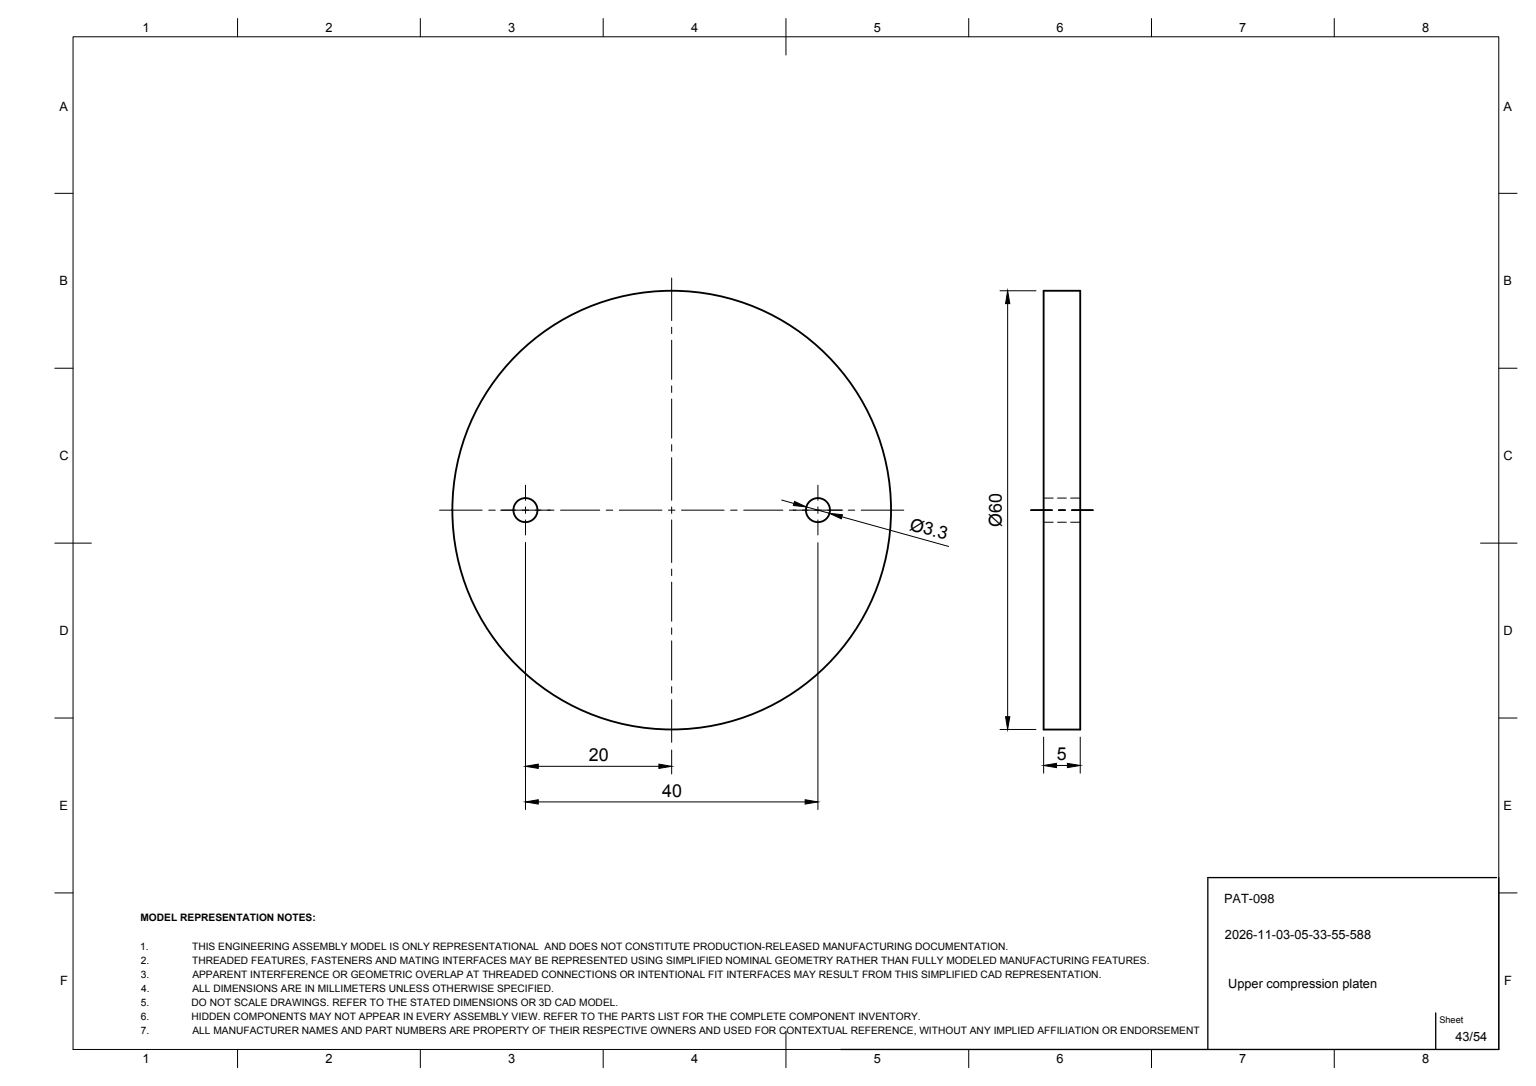
ISO-10303-21;
HEADER;
/* Generated by software containing ST-Developer
 * from STEP Tools, Inc. (www.steptools.com) 
 */

FILE_DESCRIPTION(
/* description */ ('Spring compression tester'),
/* implementation_level */ '2;1');

FILE_NAME(
/* name */ 'Upper compression platen.step',
/* time_stamp */ '2026-10-28T03:24:11-07:00',
/* author */ (''),
/* organization */ (''),
/* preprocessor_version */ 'ST-DEVELOPER v20.2',
/* originating_system */ 'Autodesk Translation Framework v15.17.0.0',
/* authorisation */ '');

FILE_SCHEMA (('AUTOMOTIVE_DESIGN { 1 0 10303 214 3 1 1 }'));
ENDSEC;

DATA;
#10=MECHANICAL_DESIGN_GEOMETRIC_PRESENTATION_REPRESENTATION('',(#1162),#43521);
#1027=SHAPE_REPRESENTATION_RELATIONSHIP('SRR','None',#43842,#1087);
#1087=ADVANCED_BREP_SHAPE_REPRESENTATION('',(#1233),#43502);
#1162=STYLED_ITEM('',(#44216),#1233);
#1233=MANIFOLD_SOLID_BREP('Body1',#18603);
#1534=FACE_BOUND('',#4226,.T.);
#1535=FACE_BOUND('',#4227,.T.);
#1536=FACE_BOUND('',#4229,.T.);
#1537=FACE_BOUND('',#4230,.T.);
#2051=PLANE('',#20617);
#2052=PLANE('',#20618);
#2888=FACE_OUTER_BOUND('',#4222,.T.);
#2889=FACE_OUTER_BOUND('',#4223,.T.);
#2890=FACE_OUTER_BOUND('',#4224,.T.);
#2891=FACE_OUTER_BOUND('',#4225,.T.);
#2892=FACE_OUTER_BOUND('',#4228,.T.);
#4222=EDGE_LOOP('',(#15483,#15484,#15485,#15486));
#4223=EDGE_LOOP('',(#15487,#15488,#15489,#15490));
#4224=EDGE_LOOP('',(#15491,#15492,#15493,#15494));
#4225=EDGE_LOOP('',(#15495));
#4226=EDGE_LOOP('',(#15496));
#4227=EDGE_LOOP('',(#15497));
#4228=EDGE_LOOP('',(#15498));
#4229=EDGE_LOOP('',(#15499));
#4230=EDGE_LOOP('',(#15500));
#5660=LINE('',#30598,#7092);
#5661=LINE('',#30604,#7093);
#5662=LINE('',#30610,#7094);
#7092=VECTOR('',#24902,0.165);
#7093=VECTOR('',#24909,0.165);
#7094=VECTOR('',#24916,3.);
#8015=CIRCLE('',#20609,0.165);
#8016=CIRCLE('',#20610,0.165);
#8017=CIRCLE('',#20612,0.165);
#8018=CIRCLE('',#20613,0.165);
#8019=CIRCLE('',#20615,3.);
#8020=CIRCLE('',#20616,3.);
#9236=VERTEX_POINT('',#30595);
#9237=VERTEX_POINT('',#30597);
#9238=VERTEX_POINT('',#30601);
#9239=VERTEX_POINT('',#30603);
#9240=VERTEX_POINT('',#30607);
#9241=VERTEX_POINT('',#30609);
#11406=EDGE_CURVE('',#9236,#9236,#8015,.T.);
#11407=EDGE_CURVE('',#9236,#9237,#5660,.T.);
#11408=EDGE_CURVE('',#9237,#9237,#8016,.T.);
#11409=EDGE_CURVE('',#9238,#9238,#8017,.T.);
#11410=EDGE_CURVE('',#9238,#9239,#5661,.T.);
#11411=EDGE_CURVE('',#9239,#9239,#8018,.T.);
#11412=EDGE_CURVE('',#9240,#9240,#8019,.T.);
#11413=EDGE_CURVE('',#9240,#9241,#5662,.T.);
#11414=EDGE_CURVE('',#9241,#9241,#8020,.T.);
#15483=ORIENTED_EDGE('',*,*,#11406,.F.);
#15484=ORIENTED_EDGE('',*,*,#11407,.T.);
#15485=ORIENTED_EDGE('',*,*,#11408,.F.);
#15486=ORIENTED_EDGE('',*,*,#11407,.F.);
#15487=ORIENTED_EDGE('',*,*,#11409,.F.);
#15488=ORIENTED_EDGE('',*,*,#11410,.T.);
#15489=ORIENTED_EDGE('',*,*,#11411,.F.);
#15490=ORIENTED_EDGE('',*,*,#11410,.F.);
#15491=ORIENTED_EDGE('',*,*,#11412,.F.);
#15492=ORIENTED_EDGE('',*,*,#11413,.T.);
#15493=ORIENTED_EDGE('',*,*,#11414,.T.);
#15494=ORIENTED_EDGE('',*,*,#11413,.F.);
#15495=ORIENTED_EDGE('',*,*,#11412,.T.);
#15496=ORIENTED_EDGE('',*,*,#11408,.T.);
#15497=ORIENTED_EDGE('',*,*,#11411,.T.);
#15498=ORIENTED_EDGE('',*,*,#11414,.F.);
#15499=ORIENTED_EDGE('',*,*,#11406,.T.);
#15500=ORIENTED_EDGE('',*,*,#11409,.T.);
#17301=CYLINDRICAL_SURFACE('',#20608,0.165);
#17302=CYLINDRICAL_SURFACE('',#20611,0.165);
#17303=CYLINDRICAL_SURFACE('',#20614,3.);
#18212=ADVANCED_FACE('',(#2888),#17301,.F.);
#18213=ADVANCED_FACE('',(#2889),#17302,.F.);
#18214=ADVANCED_FACE('',(#2890),#17303,.T.);
#18215=ADVANCED_FACE('',(#2891,#1534,#1535),#2051,.T.);
#18216=ADVANCED_FACE('',(#2892,#1536,#1537),#2052,.F.);
#18603=CLOSED_SHELL('',(#18212,#18213,#18214,#18215,#18216));
#20607=AXIS2_PLACEMENT_3D('',#30593,#24896,#24897);
#20608=AXIS2_PLACEMENT_3D('',#30594,#24898,#24899);
#20609=AXIS2_PLACEMENT_3D('',#30596,#24900,#24901);
#20610=AXIS2_PLACEMENT_3D('',#30599,#24903,#24904);
#20611=AXIS2_PLACEMENT_3D('',#30600,#24905,#24906);
#20612=AXIS2_PLACEMENT_3D('',#30602,#24907,#24908);
#20613=AXIS2_PLACEMENT_3D('',#30605,#24910,#24911);
#20614=AXIS2_PLACEMENT_3D('',#30606,#24912,#24913);
#20615=AXIS2_PLACEMENT_3D('',#30608,#24914,#24915);
#20616=AXIS2_PLACEMENT_3D('',#30611,#24917,#24918);
#20617=AXIS2_PLACEMENT_3D('',#30612,#24919,#24920);
#20618=AXIS2_PLACEMENT_3D('',#30613,#24921,#24922);
#24896=DIRECTION('axis',(0.,0.,1.));
#24897=DIRECTION('refdir',(1.,0.,0.));
#24898=DIRECTION('center_axis',(0.,0.,1.));
#24899=DIRECTION('ref_axis',(1.,0.,0.));
#24900=DIRECTION('center_axis',(0.,0.,1.));
#24901=DIRECTION('ref_axis',(1.,0.,0.));
#24902=DIRECTION('',(0.,0.,1.));
#24903=DIRECTION('center_axis',(0.,0.,-1.));
#24904=DIRECTION('ref_axis',(1.,0.,0.));
#24905=DIRECTION('center_axis',(0.,0.,1.));
#24906=DIRECTION('ref_axis',(1.,0.,0.));
#24907=DIRECTION('center_axis',(0.,0.,1.));
#24908=DIRECTION('ref_axis',(1.,0.,0.));
#24909=DIRECTION('',(0.,0.,1.));
#24910=DIRECTION('center_axis',(0.,0.,-1.));
#24911=DIRECTION('ref_axis',(1.,0.,0.));
#24912=DIRECTION('center_axis',(0.,0.,1.));
#24913=DIRECTION('ref_axis',(1.,0.,0.));
#24914=DIRECTION('center_axis',(0.,0.,1.));
#24915=DIRECTION('ref_axis',(1.,0.,0.));
#24916=DIRECTION('',(0.,0.,-1.));
#24917=DIRECTION('center_axis',(0.,0.,1.));
#24918=DIRECTION('ref_axis',(1.,0.,0.));
#24919=DIRECTION('center_axis',(0.,0.,1.));
#24920=DIRECTION('ref_axis',(1.,0.,0.));
#24921=DIRECTION('center_axis',(0.,0.,1.));
#24922=DIRECTION('ref_axis',(1.,0.,0.));
#30593=CARTESIAN_POINT('',(0.,0.,0.));
#30594=CARTESIAN_POINT('Origin',(-2.,-1.5,14.5));
#30595=CARTESIAN_POINT('',(-2.165,-1.5,14.6));
#30596=CARTESIAN_POINT('Origin',(-2.,-1.5,14.6));
#30597=CARTESIAN_POINT('',(-2.165,-1.5,15.1));
#30598=CARTESIAN_POINT('',(-2.165,-1.5,14.5));
#30599=CARTESIAN_POINT('Origin',(-2.,-1.5,15.1));
#30600=CARTESIAN_POINT('Origin',(2.,-1.5,14.5));
#30601=CARTESIAN_POINT('',(1.835,-1.5,14.6));
#30602=CARTESIAN_POINT('Origin',(2.,-1.5,14.6));
#30603=CARTESIAN_POINT('',(1.835,-1.5,15.1));
#30604=CARTESIAN_POINT('',(1.835,-1.5,14.5));
#30605=CARTESIAN_POINT('Origin',(2.,-1.5,15.1));
#30606=CARTESIAN_POINT('Origin',(0.,-1.5,14.6));
#30607=CARTESIAN_POINT('',(-3.,-1.5,15.1));
#30608=CARTESIAN_POINT('Origin',(0.,-1.5,15.1));
#30609=CARTESIAN_POINT('',(-3.,-1.5,14.6));
#30610=CARTESIAN_POINT('',(-3.,-1.5,14.6));
#30611=CARTESIAN_POINT('Origin',(0.,-1.5,14.6));
#30612=CARTESIAN_POINT('Origin',(0.,-1.5,15.1));
#30613=CARTESIAN_POINT('Origin',(0.,-1.5,14.6));
#43434=UNCERTAINTY_MEASURE_WITH_UNIT(LENGTH_MEASURE(0.001),#43522,
'DISTANCE_ACCURACY_VALUE',
'Maximum model space distance between geometric entities at asserted c
onnectivities');
#43453=UNCERTAINTY_MEASURE_WITH_UNIT(LENGTH_MEASURE(0.001),#43522,
'DISTANCE_ACCURACY_VALUE',
'Maximum model space distance between geometric entities at asserted c
onnectivities');
#43502=(
GEOMETRIC_REPRESENTATION_CONTEXT(3)
GLOBAL_UNCERTAINTY_ASSIGNED_CONTEXT((#43434))
GLOBAL_UNIT_ASSIGNED_CONTEXT((#43522,#43524,#43525))
REPRESENTATION_CONTEXT('','3D')
);
#43521=(
GEOMETRIC_REPRESENTATION_CONTEXT(3)
GLOBAL_UNCERTAINTY_ASSIGNED_CONTEXT((#43453))
GLOBAL_UNIT_ASSIGNED_CONTEXT((#43522,#43524,#43525))
REPRESENTATION_CONTEXT('','3D')
);
#43522=(
LENGTH_UNIT()
NAMED_UNIT(*)
SI_UNIT(.CENTI.,.METRE.)
);
#43524=(
NAMED_UNIT(*)
PLANE_ANGLE_UNIT()
SI_UNIT($,.RADIAN.)
);
#43525=(
NAMED_UNIT(*)
SI_UNIT($,.STERADIAN.)
SOLID_ANGLE_UNIT()
);
#43574=SHAPE_DEFINITION_REPRESENTATION(#43651,#43842);
#43651=PRODUCT_DEFINITION_SHAPE('',$,#43910);
#43842=SHAPE_REPRESENTATION('',(#20607),#43502);
#43861=PRODUCT_DEFINITION_CONTEXT('part definition',#44064,'design');
#43910=PRODUCT_DEFINITION('Upper compression platen',
'Upper compression platen',#43977,#43861);
#43977=PRODUCT_DEFINITION_FORMATION('',$,#44114);
#44064=APPLICATION_CONTEXT(
'Core Data for Automotive Mechanical Design Process');
#44065=PRODUCT_CONTEXT('part definition',#44064,'mechanical');
#44114=PRODUCT('Upper compression platen','Upper compression platen',
'Upper compression platen',(#44065));
#44210=COLOUR_RGB('Off White',0.89,0.88,0.83);
#44211=FILL_AREA_STYLE_COLOUR('',#44210);
#44212=FILL_AREA_STYLE('',(#44211));
#44213=SURFACE_STYLE_FILL_AREA(#44212);
#44214=SURFACE_SIDE_STYLE('',(#44213));
#44215=SURFACE_STYLE_USAGE(.BOTH.,#44214);
#44216=PRESENTATION_STYLE_ASSIGNMENT((#44215));
ENDSEC;
END-ISO-10303-21;
